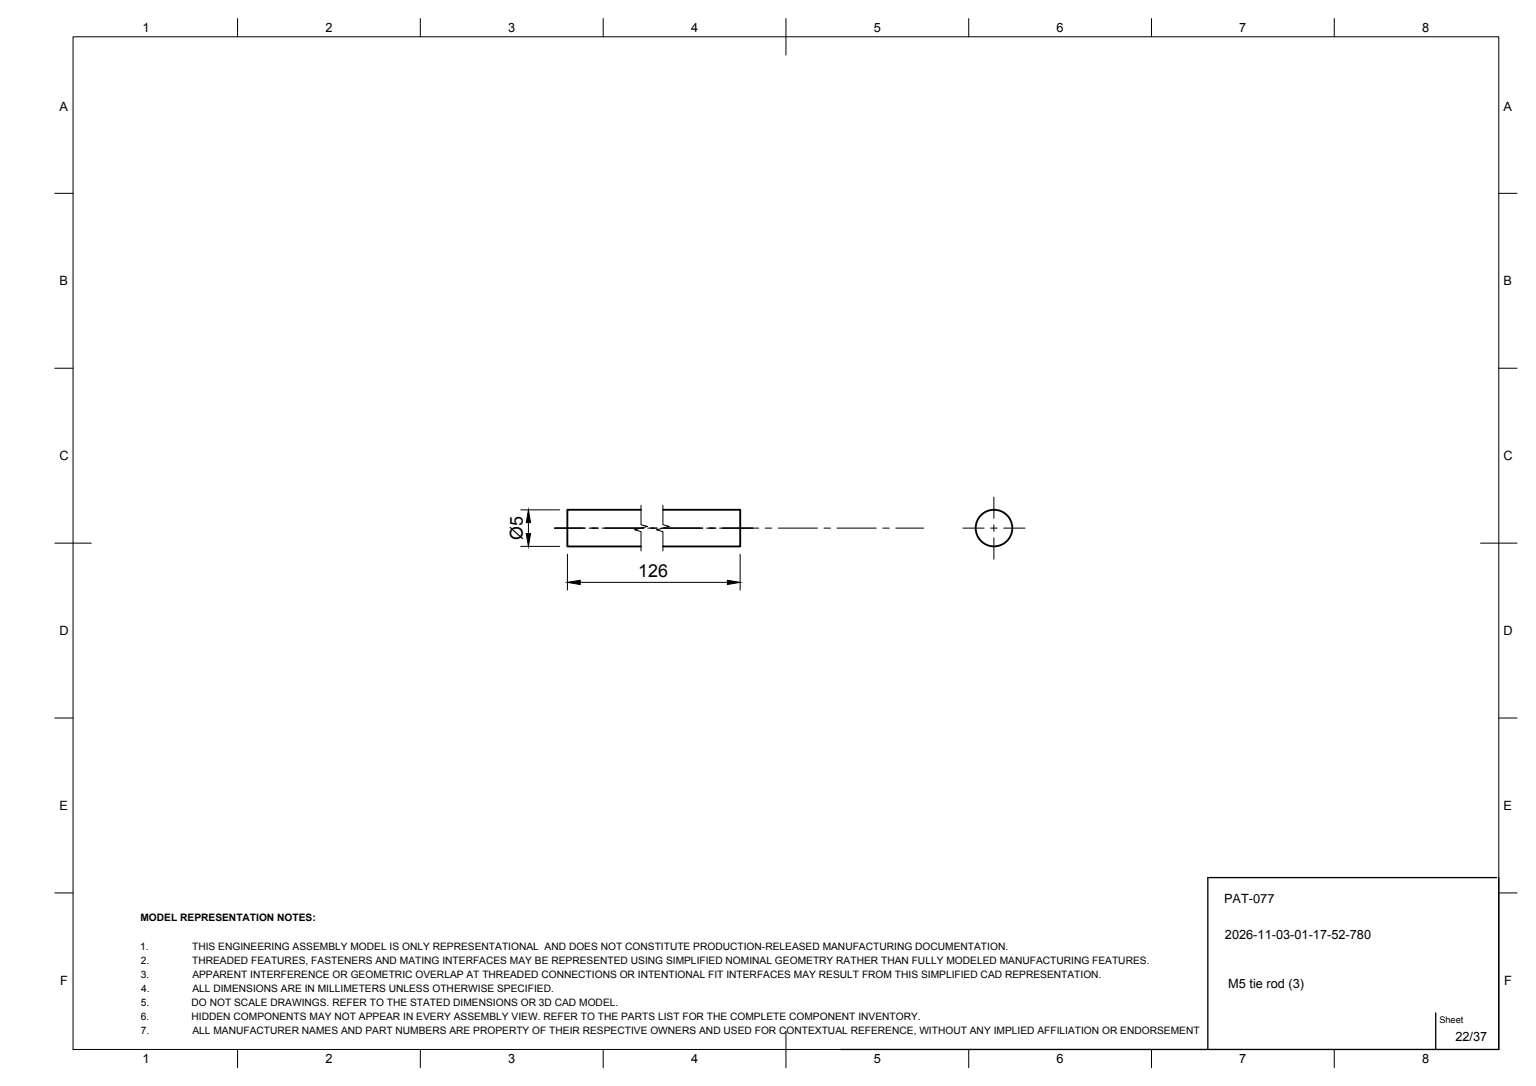
ISO-10303-21;
HEADER;
/* Generated by software containing ST-Developer
 * from STEP Tools, Inc. (www.steptools.com) 
 */

FILE_DESCRIPTION(
/* description */ ('Pallet stop with pneumatic fitting'),
/* implementation_level */ '2;1');

FILE_NAME(
/* name */ 'M5 tie rod (3).step',
/* time_stamp */ '2026-10-27T10:51:41-07:00',
/* author */ (''),
/* organization */ (''),
/* preprocessor_version */ 'ST-DEVELOPER v20.2',
/* originating_system */ 'Autodesk Translation Framework v15.17.0.0',
/* authorisation */ '');

FILE_SCHEMA (('AUTOMOTIVE_DESIGN { 1 0 10303 214 3 1 1 }'));
ENDSEC;

DATA;
#10=MECHANICAL_DESIGN_GEOMETRIC_PRESENTATION_REPRESENTATION('',(#374),#10265);
#310=SHAPE_REPRESENTATION_RELATIONSHIP('SRR','None',#10423,#342);
#342=ADVANCED_BREP_SHAPE_REPRESENTATION('',(#406),#10247);
#374=STYLED_ITEM('',(#10655),#406);
#406=MANIFOLD_SOLID_BREP('Body1',#5062);
#630=PLANE('',#5749);
#631=PLANE('',#5750);
#891=FACE_OUTER_BOUND('',#1290,.T.);
#892=FACE_OUTER_BOUND('',#1291,.T.);
#893=FACE_OUTER_BOUND('',#1292,.T.);
#1290=EDGE_LOOP('',(#3994,#3995,#3996,#3997));
#1291=EDGE_LOOP('',(#3998));
#1292=EDGE_LOOP('',(#3999));
#1635=LINE('',#9355,#1970);
#1970=VECTOR('',#6866,0.25);
#2300=CIRCLE('',#5747,0.25);
#2301=CIRCLE('',#5748,0.25);
#2600=VERTEX_POINT('',#9352);
#2601=VERTEX_POINT('',#9354);
#3096=EDGE_CURVE('',#2600,#2600,#2300,.T.);
#3097=EDGE_CURVE('',#2600,#2601,#1635,.T.);
#3098=EDGE_CURVE('',#2601,#2601,#2301,.T.);
#3994=ORIENTED_EDGE('',*,*,#3096,.F.);
#3995=ORIENTED_EDGE('',*,*,#3097,.T.);
#3996=ORIENTED_EDGE('',*,*,#3098,.T.);
#3997=ORIENTED_EDGE('',*,*,#3097,.F.);
#3998=ORIENTED_EDGE('',*,*,#3096,.T.);
#3999=ORIENTED_EDGE('',*,*,#3098,.F.);
#4691=CYLINDRICAL_SURFACE('',#5746,0.25);
#4886=ADVANCED_FACE('',(#891),#4691,.T.);
#4887=ADVANCED_FACE('',(#892),#630,.T.);
#4888=ADVANCED_FACE('',(#893),#631,.F.);
#5062=CLOSED_SHELL('',(#4886,#4887,#4888));
#5745=AXIS2_PLACEMENT_3D('',#9350,#6860,#6861);
#5746=AXIS2_PLACEMENT_3D('',#9351,#6862,#6863);
#5747=AXIS2_PLACEMENT_3D('',#9353,#6864,#6865);
#5748=AXIS2_PLACEMENT_3D('',#9356,#6867,#6868);
#5749=AXIS2_PLACEMENT_3D('',#9357,#6869,#6870);
#5750=AXIS2_PLACEMENT_3D('',#9358,#6871,#6872);
#6860=DIRECTION('axis',(0.,0.,1.));
#6861=DIRECTION('refdir',(1.,0.,0.));
#6862=DIRECTION('center_axis',(0.,0.,1.));
#6863=DIRECTION('ref_axis',(1.,0.,0.));
#6864=DIRECTION('center_axis',(0.,0.,1.));
#6865=DIRECTION('ref_axis',(1.,0.,0.));
#6866=DIRECTION('',(0.,0.,-1.));
#6867=DIRECTION('center_axis',(0.,0.,1.));
#6868=DIRECTION('ref_axis',(1.,0.,0.));
#6869=DIRECTION('center_axis',(0.,0.,1.));
#6870=DIRECTION('ref_axis',(1.,0.,0.));
#6871=DIRECTION('center_axis',(0.,0.,1.));
#6872=DIRECTION('ref_axis',(1.,0.,0.));
#9350=CARTESIAN_POINT('',(0.,0.,0.));
#9351=CARTESIAN_POINT('Origin',(5.27279220613578,2.72720779386421,-1.8));
#9352=CARTESIAN_POINT('',(5.02279220613578,2.72720779386421,10.8));
#9353=CARTESIAN_POINT('Origin',(5.27279220613578,2.72720779386421,10.8));
#9354=CARTESIAN_POINT('',(5.02279220613578,2.72720779386421,-1.8));
#9355=CARTESIAN_POINT('',(5.02279220613578,2.72720779386421,-1.8));
#9356=CARTESIAN_POINT('Origin',(5.27279220613578,2.72720779386421,-1.8));
#9357=CARTESIAN_POINT('Origin',(5.27279220613578,2.72720779386421,10.8));
#9358=CARTESIAN_POINT('Origin',(5.27279220613578,2.72720779386421,-1.8));
#10209=UNCERTAINTY_MEASURE_WITH_UNIT(LENGTH_MEASURE(0.001),#10266,
'DISTANCE_ACCURACY_VALUE',
'Maximum model space distance between geometric entities at asserted c
onnectivities');
#10227=UNCERTAINTY_MEASURE_WITH_UNIT(LENGTH_MEASURE(0.001),#10266,
'DISTANCE_ACCURACY_VALUE',
'Maximum model space distance between geometric entities at asserted c
onnectivities');
#10247=(
GEOMETRIC_REPRESENTATION_CONTEXT(3)
GLOBAL_UNCERTAINTY_ASSIGNED_CONTEXT((#10209))
GLOBAL_UNIT_ASSIGNED_CONTEXT((#10266,#10268,#10269))
REPRESENTATION_CONTEXT('','3D')
);
#10265=(
GEOMETRIC_REPRESENTATION_CONTEXT(3)
GLOBAL_UNCERTAINTY_ASSIGNED_CONTEXT((#10227))
GLOBAL_UNIT_ASSIGNED_CONTEXT((#10266,#10268,#10269))
REPRESENTATION_CONTEXT('','3D')
);
#10266=(
LENGTH_UNIT()
NAMED_UNIT(*)
SI_UNIT(.CENTI.,.METRE.)
);
#10268=(
NAMED_UNIT(*)
PLANE_ANGLE_UNIT()
SI_UNIT($,.RADIAN.)
);
#10269=(
NAMED_UNIT(*)
SI_UNIT($,.STERADIAN.)
SOLID_ANGLE_UNIT()
);
#10289=SHAPE_DEFINITION_REPRESENTATION(#10326,#10423);
#10326=PRODUCT_DEFINITION_SHAPE('',$,#10461);
#10423=SHAPE_REPRESENTATION('',(#5745),#10247);
#10441=PRODUCT_DEFINITION_CONTEXT('part definition',#10554,'design');
#10461=PRODUCT_DEFINITION('M5 tie rod (3)','M5 tie rod (3)',#10498,#10441);
#10498=PRODUCT_DEFINITION_FORMATION('',$,#10575);
#10554=APPLICATION_CONTEXT(
'Core Data for Automotive Mechanical Design Process');
#10555=PRODUCT_CONTEXT('part definition',#10554,'mechanical');
#10575=PRODUCT('M5 tie rod (3)','M5 tie rod (3)','M5 tie rod (3)',(#10555));
#10649=COLOUR_RGB('Grey',0.48,0.52,0.57);
#10650=FILL_AREA_STYLE_COLOUR('',#10649);
#10651=FILL_AREA_STYLE('',(#10650));
#10652=SURFACE_STYLE_FILL_AREA(#10651);
#10653=SURFACE_SIDE_STYLE('',(#10652));
#10654=SURFACE_STYLE_USAGE(.BOTH.,#10653);
#10655=PRESENTATION_STYLE_ASSIGNMENT((#10654));
ENDSEC;
END-ISO-10303-21;
